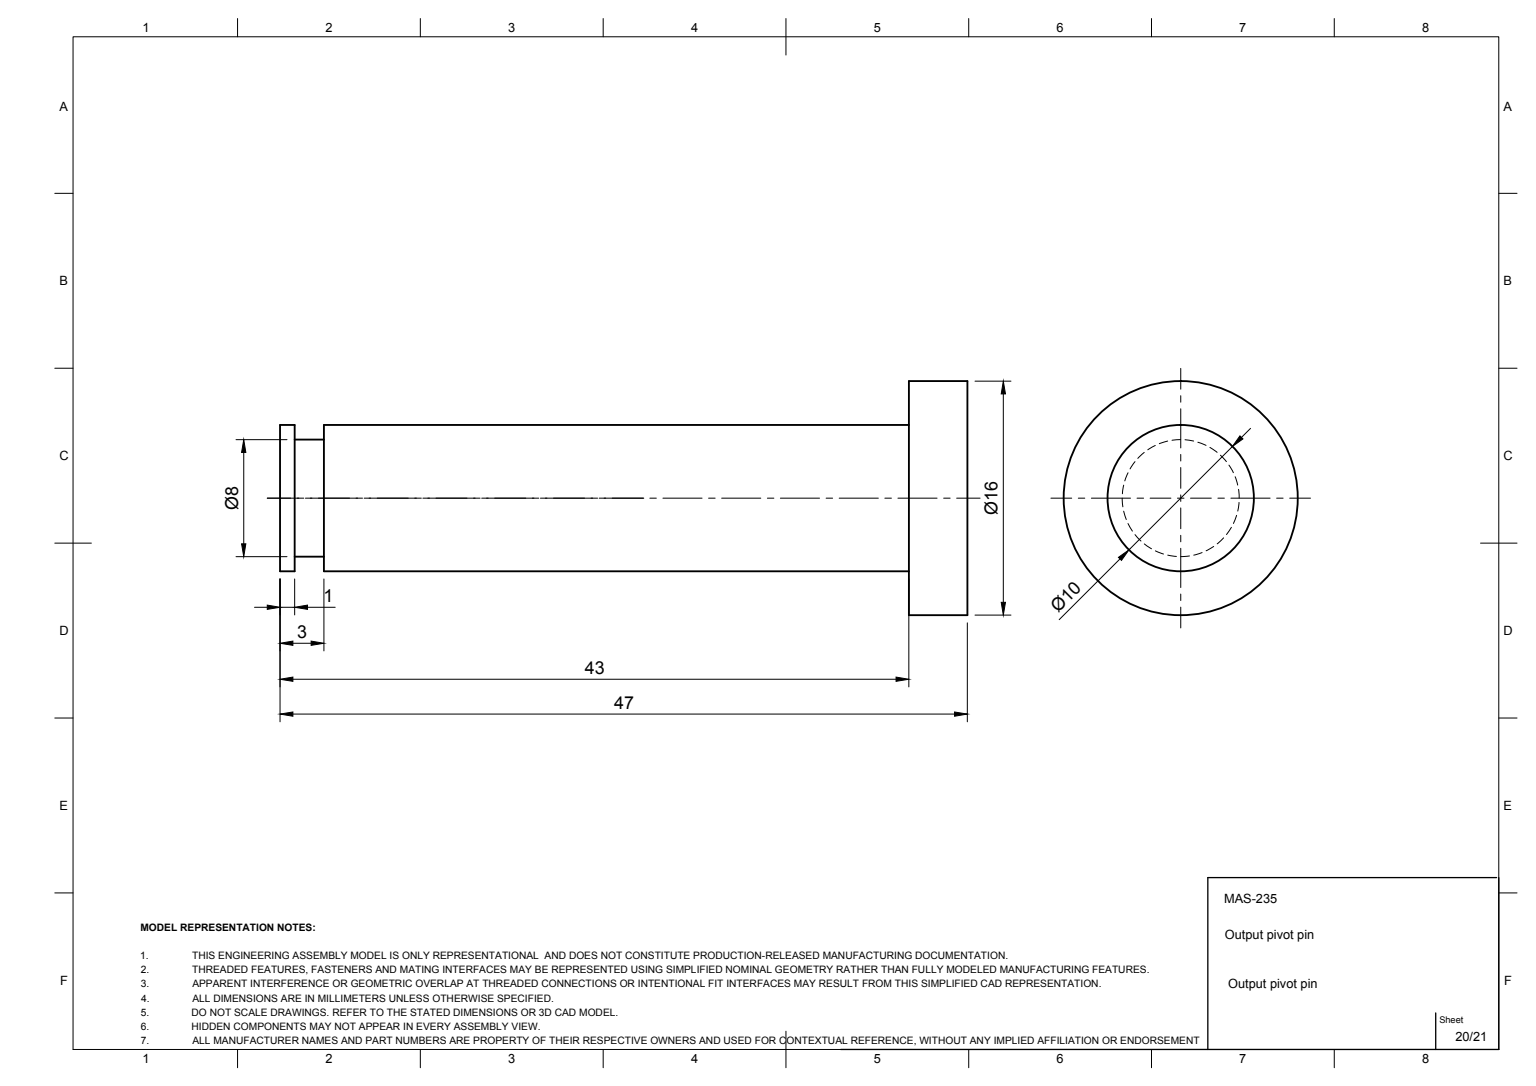
ISO-10303-21;
HEADER;
/* Generated by software containing ST-Developer
 * from STEP Tools, Inc. (www.steptools.com) 
 */

FILE_DESCRIPTION(
/* description */ ('Independent Whitworth quick-return mechanism. Crank radius40, ground-
center spacing80, lever180, connecting rod160, output guide X200. Nomi
nal stroke180 and long/short phase ratio2. Retained guide rods, replac
eable bearing sleeves and captured sliding shoe. No load or production
 rating assigned.'),
/* implementation_level */ '2;1');

FILE_NAME(
/* name */ 'Output pivot pin.step',
/* time_stamp */ '2026-11-09T18:22:56-08:00',
/* author */ (''),
/* organization */ (''),
/* preprocessor_version */ 'ST-DEVELOPER v20.2',
/* originating_system */ 'Autodesk Translation Framework v15.17.0.0',
/* authorisation */ '');

FILE_SCHEMA (('AUTOMOTIVE_DESIGN { 1 0 10303 214 3 1 1 }'));
ENDSEC;

DATA;
#10=MECHANICAL_DESIGN_GEOMETRIC_PRESENTATION_REPRESENTATION('',(#234),#4388);
#194=SHAPE_REPRESENTATION_RELATIONSHIP('SRR','None',#4493,#214);
#214=ADVANCED_BREP_SHAPE_REPRESENTATION('',(#254),#4383);
#234=STYLED_ITEM('',(#4595),#254);
#254=MANIFOLD_SOLID_BREP('Body1',#2339);
#310=FACE_BOUND('',#725,.T.);
#311=FACE_BOUND('',#727,.T.);
#312=FACE_BOUND('',#730,.T.);
#390=PLANE('',#2803);
#391=PLANE('',#2805);
#392=PLANE('',#2809);
#393=PLANE('',#2814);
#394=PLANE('',#2816);
#525=FACE_OUTER_BOUND('',#723,.T.);
#526=FACE_OUTER_BOUND('',#724,.T.);
#527=FACE_OUTER_BOUND('',#726,.T.);
#528=FACE_OUTER_BOUND('',#728,.T.);
#529=FACE_OUTER_BOUND('',#729,.T.);
#530=FACE_OUTER_BOUND('',#731,.T.);
#531=FACE_OUTER_BOUND('',#732,.T.);
#532=FACE_OUTER_BOUND('',#733,.T.);
#533=FACE_OUTER_BOUND('',#734,.T.);
#723=EDGE_LOOP('',(#2032,#2033,#2034,#2035));
#724=EDGE_LOOP('',(#2036));
#725=EDGE_LOOP('',(#2037));
#726=EDGE_LOOP('',(#2038));
#727=EDGE_LOOP('',(#2039));
#728=EDGE_LOOP('',(#2040,#2041,#2042,#2043));
#729=EDGE_LOOP('',(#2044));
#730=EDGE_LOOP('',(#2045));
#731=EDGE_LOOP('',(#2046,#2047,#2048,#2049));
#732=EDGE_LOOP('',(#2050));
#733=EDGE_LOOP('',(#2051,#2052,#2053,#2054));
#734=EDGE_LOOP('',(#2055));
#880=LINE('',#4206,#1019);
#881=LINE('',#4217,#1020);
#882=LINE('',#4225,#1021);
#883=LINE('',#4229,#1022);
#1019=VECTOR('',#3492,4.);
#1020=VECTOR('',#3507,5.);
#1021=VECTOR('',#3516,8.);
#1022=VECTOR('',#3523,5.);
#1135=CIRCLE('',#2801,4.);
#1136=CIRCLE('',#2802,4.);
#1137=CIRCLE('',#2804,5.);
#1138=CIRCLE('',#2806,5.);
#1139=CIRCLE('',#2808,5.);
#1140=CIRCLE('',#2810,8.);
#1141=CIRCLE('',#2811,5.);
#1142=CIRCLE('',#2813,8.);
#1305=VERTEX_POINT('',#4203);
#1306=VERTEX_POINT('',#4205);
#1307=VERTEX_POINT('',#4209);
#1308=VERTEX_POINT('',#4212);
#1309=VERTEX_POINT('',#4215);
#1310=VERTEX_POINT('',#4219);
#1311=VERTEX_POINT('',#4221);
#1312=VERTEX_POINT('',#4224);
#1552=EDGE_CURVE('',#1305,#1305,#1135,.T.);
#1553=EDGE_CURVE('',#1305,#1306,#880,.T.);
#1554=EDGE_CURVE('',#1306,#1306,#1136,.T.);
#1555=EDGE_CURVE('',#1307,#1307,#1137,.T.);
#1556=EDGE_CURVE('',#1308,#1308,#1138,.T.);
#1557=EDGE_CURVE('',#1309,#1309,#1139,.T.);
#1558=EDGE_CURVE('',#1309,#1308,#881,.T.);
#1559=EDGE_CURVE('',#1310,#1310,#1140,.T.);
#1560=EDGE_CURVE('',#1311,#1311,#1141,.T.);
#1561=EDGE_CURVE('',#1310,#1312,#882,.T.);
#1562=EDGE_CURVE('',#1312,#1312,#1142,.T.);
#1563=EDGE_CURVE('',#1307,#1311,#883,.T.);
#2032=ORIENTED_EDGE('',*,*,#1552,.T.);
#2033=ORIENTED_EDGE('',*,*,#1553,.T.);
#2034=ORIENTED_EDGE('',*,*,#1554,.F.);
#2035=ORIENTED_EDGE('',*,*,#1553,.F.);
#2036=ORIENTED_EDGE('',*,*,#1555,.F.);
#2037=ORIENTED_EDGE('',*,*,#1552,.F.);
#2038=ORIENTED_EDGE('',*,*,#1556,.F.);
#2039=ORIENTED_EDGE('',*,*,#1554,.T.);
#2040=ORIENTED_EDGE('',*,*,#1557,.F.);
#2041=ORIENTED_EDGE('',*,*,#1558,.T.);
#2042=ORIENTED_EDGE('',*,*,#1556,.T.);
#2043=ORIENTED_EDGE('',*,*,#1558,.F.);
#2044=ORIENTED_EDGE('',*,*,#1559,.T.);
#2045=ORIENTED_EDGE('',*,*,#1560,.F.);
#2046=ORIENTED_EDGE('',*,*,#1559,.F.);
#2047=ORIENTED_EDGE('',*,*,#1561,.T.);
#2048=ORIENTED_EDGE('',*,*,#1562,.T.);
#2049=ORIENTED_EDGE('',*,*,#1561,.F.);
#2050=ORIENTED_EDGE('',*,*,#1562,.F.);
#2051=ORIENTED_EDGE('',*,*,#1555,.T.);
#2052=ORIENTED_EDGE('',*,*,#1563,.T.);
#2053=ORIENTED_EDGE('',*,*,#1560,.T.);
#2054=ORIENTED_EDGE('',*,*,#1563,.F.);
#2055=ORIENTED_EDGE('',*,*,#1557,.T.);
#2165=CYLINDRICAL_SURFACE('',#2800,4.);
#2166=CYLINDRICAL_SURFACE('',#2807,5.);
#2167=CYLINDRICAL_SURFACE('',#2812,8.);
#2168=CYLINDRICAL_SURFACE('',#2815,5.);
#2297=ADVANCED_FACE('',(#525),#2165,.T.);
#2298=ADVANCED_FACE('',(#526,#310),#390,.F.);
#2299=ADVANCED_FACE('',(#527,#311),#391,.F.);
#2300=ADVANCED_FACE('',(#528),#2166,.T.);
#2301=ADVANCED_FACE('',(#529,#312),#392,.T.);
#2302=ADVANCED_FACE('',(#530),#2167,.T.);
#2303=ADVANCED_FACE('',(#531),#393,.F.);
#2304=ADVANCED_FACE('',(#532),#2168,.T.);
#2305=ADVANCED_FACE('',(#533),#394,.T.);
#2339=CLOSED_SHELL('',(#2297,#2298,#2299,#2300,#2301,#2302,#2303,#2304,
#2305));
#2799=AXIS2_PLACEMENT_3D('',#4201,#3486,#3487);
#2800=AXIS2_PLACEMENT_3D('',#4202,#3488,#3489);
#2801=AXIS2_PLACEMENT_3D('',#4204,#3490,#3491);
#2802=AXIS2_PLACEMENT_3D('',#4207,#3493,#3494);
#2803=AXIS2_PLACEMENT_3D('',#4208,#3495,#3496);
#2804=AXIS2_PLACEMENT_3D('',#4210,#3497,#3498);
#2805=AXIS2_PLACEMENT_3D('',#4211,#3499,#3500);
#2806=AXIS2_PLACEMENT_3D('',#4213,#3501,#3502);
#2807=AXIS2_PLACEMENT_3D('',#4214,#3503,#3504);
#2808=AXIS2_PLACEMENT_3D('',#4216,#3505,#3506);
#2809=AXIS2_PLACEMENT_3D('',#4218,#3508,#3509);
#2810=AXIS2_PLACEMENT_3D('',#4220,#3510,#3511);
#2811=AXIS2_PLACEMENT_3D('',#4222,#3512,#3513);
#2812=AXIS2_PLACEMENT_3D('',#4223,#3514,#3515);
#2813=AXIS2_PLACEMENT_3D('',#4226,#3517,#3518);
#2814=AXIS2_PLACEMENT_3D('',#4227,#3519,#3520);
#2815=AXIS2_PLACEMENT_3D('',#4228,#3521,#3522);
#2816=AXIS2_PLACEMENT_3D('',#4230,#3524,#3525);
#3486=DIRECTION('axis',(0.,0.,1.));
#3487=DIRECTION('refdir',(1.,0.,0.));
#3488=DIRECTION('center_axis',(0.,0.,1.));
#3489=DIRECTION('ref_axis',(1.,0.,0.));
#3490=DIRECTION('center_axis',(0.,0.,1.));
#3491=DIRECTION('ref_axis',(1.,0.,0.));
#3492=DIRECTION('',(0.,0.,1.));
#3493=DIRECTION('center_axis',(0.,0.,1.));
#3494=DIRECTION('ref_axis',(1.,0.,0.));
#3495=DIRECTION('center_axis',(0.,0.,-1.));
#3496=DIRECTION('ref_axis',(-1.,0.,0.));
#3497=DIRECTION('center_axis',(0.,0.,-1.));
#3498=DIRECTION('ref_axis',(1.,0.,0.));
#3499=DIRECTION('center_axis',(0.,0.,1.));
#3500=DIRECTION('ref_axis',(1.,0.,0.));
#3501=DIRECTION('center_axis',(0.,0.,1.));
#3502=DIRECTION('ref_axis',(1.,0.,0.));
#3503=DIRECTION('center_axis',(0.,0.,1.));
#3504=DIRECTION('ref_axis',(1.,0.,0.));
#3505=DIRECTION('center_axis',(0.,0.,1.));
#3506=DIRECTION('ref_axis',(1.,0.,0.));
#3507=DIRECTION('',(0.,0.,-1.));
#3508=DIRECTION('center_axis',(0.,0.,1.));
#3509=DIRECTION('ref_axis',(1.,0.,0.));
#3510=DIRECTION('center_axis',(0.,0.,1.));
#3511=DIRECTION('ref_axis',(1.,0.,0.));
#3512=DIRECTION('center_axis',(0.,0.,1.));
#3513=DIRECTION('ref_axis',(1.,0.,0.));
#3514=DIRECTION('center_axis',(0.,0.,1.));
#3515=DIRECTION('ref_axis',(1.,0.,0.));
#3516=DIRECTION('',(0.,0.,-1.));
#3517=DIRECTION('center_axis',(0.,0.,1.));
#3518=DIRECTION('ref_axis',(1.,0.,0.));
#3519=DIRECTION('center_axis',(0.,0.,1.));
#3520=DIRECTION('ref_axis',(1.,0.,0.));
#3521=DIRECTION('center_axis',(0.,0.,1.));
#3522=DIRECTION('ref_axis',(1.,0.,0.));
#3523=DIRECTION('',(0.,0.,-1.));
#3524=DIRECTION('center_axis',(0.,0.,1.));
#3525=DIRECTION('ref_axis',(1.,0.,0.));
#4201=CARTESIAN_POINT('',(0.,0.,0.));
#4202=CARTESIAN_POINT('Origin',(0.,0.,41.));
#4203=CARTESIAN_POINT('',(-4.,-4.89858719658941E-16,40.));
#4204=CARTESIAN_POINT('Origin',(0.,0.,40.));
#4205=CARTESIAN_POINT('',(-4.,-4.89858719658941E-16,42.));
#4206=CARTESIAN_POINT('',(-4.,-4.89858719658941E-16,41.));
#4207=CARTESIAN_POINT('Origin',(0.,0.,42.));
#4208=CARTESIAN_POINT('Origin',(8.,0.,40.));
#4209=CARTESIAN_POINT('',(-5.,6.12323399573677E-16,40.));
#4210=CARTESIAN_POINT('Origin',(0.,0.,40.));
#4211=CARTESIAN_POINT('Origin',(4.,0.,42.));
#4212=CARTESIAN_POINT('',(-5.,-6.12323399573677E-16,42.));
#4213=CARTESIAN_POINT('Origin',(0.,0.,42.));
#4214=CARTESIAN_POINT('Origin',(0.,0.,0.));
#4215=CARTESIAN_POINT('',(-5.,-6.12323399573677E-16,43.));
#4216=CARTESIAN_POINT('Origin',(0.,0.,43.));
#4217=CARTESIAN_POINT('',(-5.,-6.12323399573677E-16,0.));
#4218=CARTESIAN_POINT('Origin',(0.,0.,0.));
#4219=CARTESIAN_POINT('',(-8.,-9.79717439317883E-16,0.));
#4220=CARTESIAN_POINT('Origin',(0.,0.,0.));
#4221=CARTESIAN_POINT('',(-5.,-6.12323399573677E-16,0.));
#4222=CARTESIAN_POINT('Origin',(0.,0.,0.));
#4223=CARTESIAN_POINT('Origin',(0.,0.,-4.));
#4224=CARTESIAN_POINT('',(-8.,-9.79717439317883E-16,-4.));
#4225=CARTESIAN_POINT('',(-8.,-9.79717439317883E-16,-4.));
#4226=CARTESIAN_POINT('Origin',(0.,0.,-4.));
#4227=CARTESIAN_POINT('Origin',(0.,0.,-4.));
#4228=CARTESIAN_POINT('Origin',(0.,0.,0.));
#4229=CARTESIAN_POINT('',(-5.,-6.12323399573677E-16,0.));
#4230=CARTESIAN_POINT('Origin',(0.,0.,43.));
#4361=UNCERTAINTY_MEASURE_WITH_UNIT(LENGTH_MEASURE(0.01),#4389,
'DISTANCE_ACCURACY_VALUE',
'Maximum model space distance between geometric entities at asserted c
onnectivities');
#4366=UNCERTAINTY_MEASURE_WITH_UNIT(LENGTH_MEASURE(0.01),#4389,
'DISTANCE_ACCURACY_VALUE',
'Maximum model space distance between geometric entities at asserted c
onnectivities');
#4383=(
GEOMETRIC_REPRESENTATION_CONTEXT(3)
GLOBAL_UNCERTAINTY_ASSIGNED_CONTEXT((#4361))
GLOBAL_UNIT_ASSIGNED_CONTEXT((#4389,#4391,#4392))
REPRESENTATION_CONTEXT('','3D')
);
#4388=(
GEOMETRIC_REPRESENTATION_CONTEXT(3)
GLOBAL_UNCERTAINTY_ASSIGNED_CONTEXT((#4366))
GLOBAL_UNIT_ASSIGNED_CONTEXT((#4389,#4391,#4392))
REPRESENTATION_CONTEXT('','3D')
);
#4389=(
LENGTH_UNIT()
NAMED_UNIT(*)
SI_UNIT(.MILLI.,.METRE.)
);
#4391=(
NAMED_UNIT(*)
PLANE_ANGLE_UNIT()
SI_UNIT($,.RADIAN.)
);
#4392=(
NAMED_UNIT(*)
SI_UNIT($,.STERADIAN.)
SOLID_ANGLE_UNIT()
);
#4409=SHAPE_DEFINITION_REPRESENTATION(#4430,#4493);
#4430=PRODUCT_DEFINITION_SHAPE('',$,#4515);
#4493=SHAPE_REPRESENTATION('',(#2799),#4383);
#4498=PRODUCT_DEFINITION_CONTEXT('part definition',#4563,'design');
#4515=PRODUCT_DEFINITION('Output pivot pin','Output pivot pin',#4536,#4498);
#4536=PRODUCT_DEFINITION_FORMATION('',$,#4581);
#4563=APPLICATION_CONTEXT(
'Core Data for Automotive Mechanical Design Process');
#4564=PRODUCT_CONTEXT('part definition',#4563,'mechanical');
#4581=PRODUCT('Output pivot pin','Output pivot pin',$,(#4564));
#4595=PRESENTATION_STYLE_ASSIGNMENT((#4609));
#4609=SURFACE_STYLE_USAGE(.BOTH.,#4623);
#4623=SURFACE_SIDE_STYLE('',(#4637));
#4637=SURFACE_STYLE_FILL_AREA(#4651);
#4651=FILL_AREA_STYLE('Pivot gray',(#4665));
#4665=FILL_AREA_STYLE_COLOUR('Pivot gray',#4679);
#4679=COLOUR_RGB('Pivot gray',0.407843137254902,0.447058823529412,0.498039215686275);
ENDSEC;
END-ISO-10303-21;
